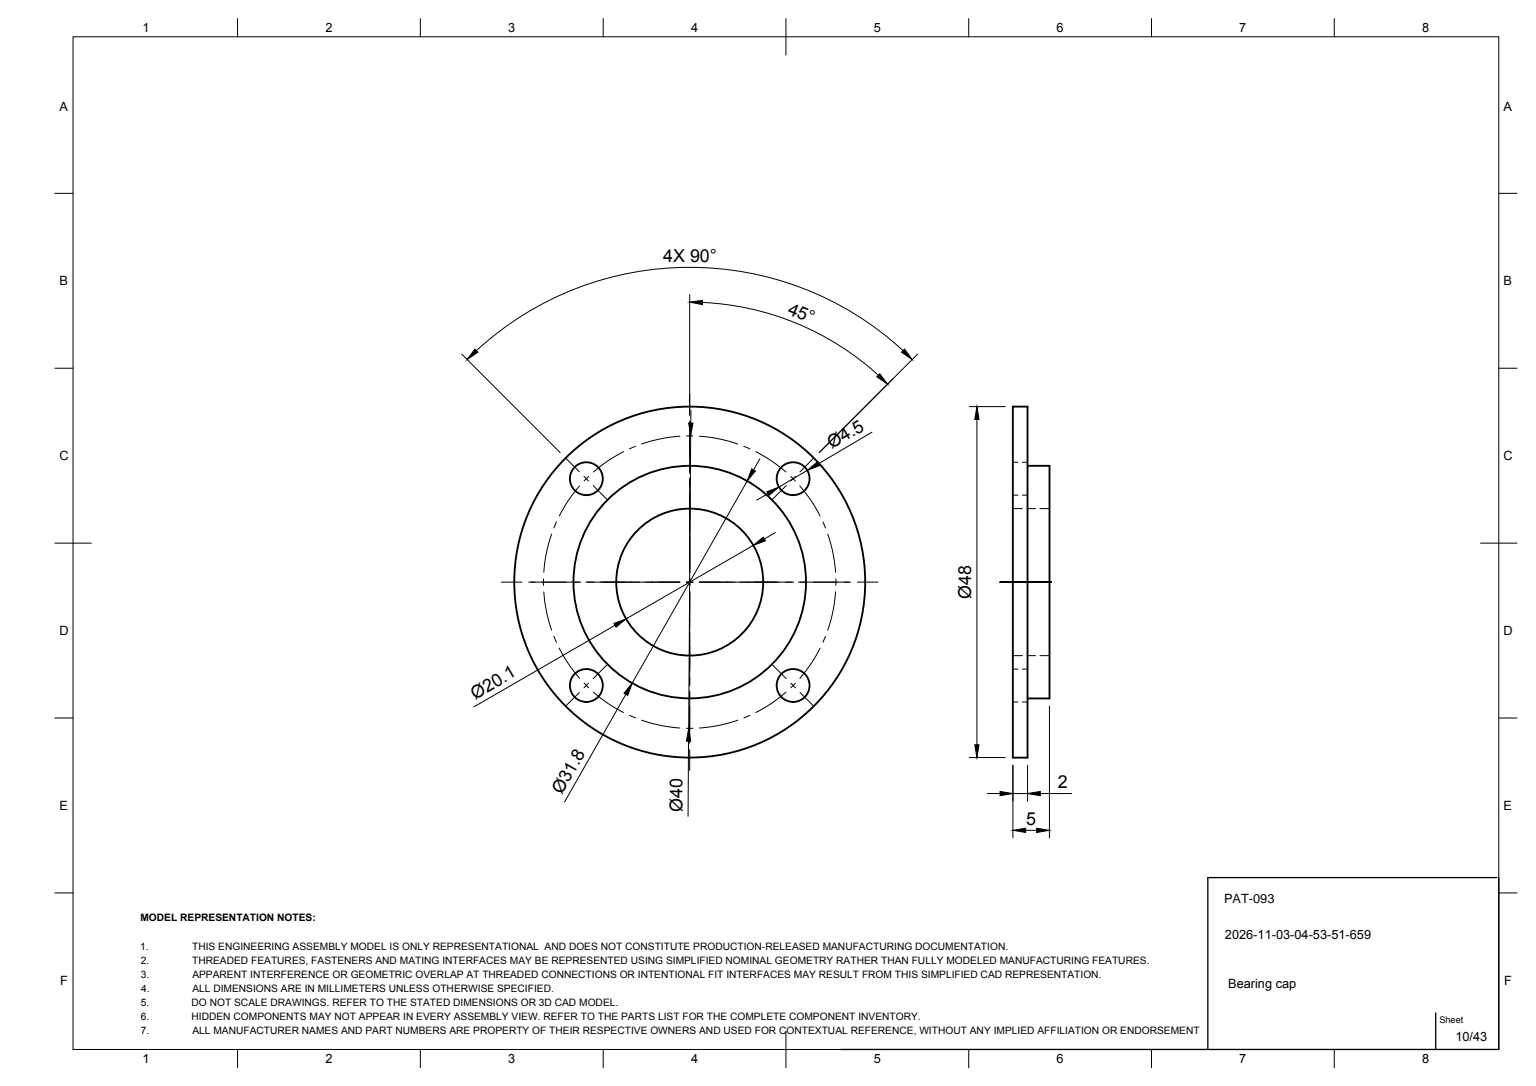
ISO-10303-21;
HEADER;
/* Generated by software containing ST-Developer
 * from STEP Tools, Inc. (www.steptools.com) 
 */

FILE_DESCRIPTION(
/* description */ ('Self-centering screw clamp'),
/* implementation_level */ '2;1');

FILE_NAME(
/* name */ 'Bearing cap.step',
/* time_stamp */ '2026-10-28T03:25:31-07:00',
/* author */ (''),
/* organization */ (''),
/* preprocessor_version */ 'ST-DEVELOPER v20.2',
/* originating_system */ 'Autodesk Translation Framework v15.17.0.0',
/* authorisation */ '');

FILE_SCHEMA (('AUTOMOTIVE_DESIGN { 1 0 10303 214 3 1 1 }'));
ENDSEC;

DATA;
#10=MECHANICAL_DESIGN_GEOMETRIC_PRESENTATION_REPRESENTATION('',(#632),#16799);
#550=SHAPE_REPRESENTATION_RELATIONSHIP('SRR','None',#17023,#591);
#591=ADVANCED_BREP_SHAPE_REPRESENTATION('',(#680),#16761);
#632=STYLED_ITEM('',(#17326),#680);
#680=MANIFOLD_SOLID_BREP('Body1',#9083);
#784=FACE_BOUND('',#1968,.T.);
#785=FACE_BOUND('',#1972,.T.);
#786=FACE_BOUND('',#1973,.T.);
#787=FACE_BOUND('',#1974,.T.);
#788=FACE_BOUND('',#1975,.T.);
#789=FACE_BOUND('',#1976,.T.);
#790=FACE_BOUND('',#1978,.T.);
#791=FACE_BOUND('',#1979,.T.);
#792=FACE_BOUND('',#1980,.T.);
#793=FACE_BOUND('',#1981,.T.);
#794=FACE_BOUND('',#1982,.T.);
#1082=PLANE('',#9828);
#1083=PLANE('',#9835);
#1084=PLANE('',#9836);
#1392=FACE_OUTER_BOUND('',#1962,.T.);
#1393=FACE_OUTER_BOUND('',#1963,.T.);
#1394=FACE_OUTER_BOUND('',#1964,.T.);
#1395=FACE_OUTER_BOUND('',#1965,.T.);
#1396=FACE_OUTER_BOUND('',#1966,.T.);
#1397=FACE_OUTER_BOUND('',#1967,.T.);
#1398=FACE_OUTER_BOUND('',#1969,.T.);
#1399=FACE_OUTER_BOUND('',#1970,.T.);
#1400=FACE_OUTER_BOUND('',#1971,.T.);
#1401=FACE_OUTER_BOUND('',#1977,.T.);
#1962=EDGE_LOOP('',(#6721,#6722,#6723,#6724));
#1963=EDGE_LOOP('',(#6725,#6726,#6727,#6728));
#1964=EDGE_LOOP('',(#6729,#6730,#6731,#6732));
#1965=EDGE_LOOP('',(#6733,#6734,#6735,#6736));
#1966=EDGE_LOOP('',(#6737,#6738,#6739,#6740));
#1967=EDGE_LOOP('',(#6741));
#1968=EDGE_LOOP('',(#6742));
#1969=EDGE_LOOP('',(#6743,#6744,#6745,#6746));
#1970=EDGE_LOOP('',(#6747,#6748,#6749,#6750));
#1971=EDGE_LOOP('',(#6751));
#1972=EDGE_LOOP('',(#6752));
#1973=EDGE_LOOP('',(#6753));
#1974=EDGE_LOOP('',(#6754));
#1975=EDGE_LOOP('',(#6755));
#1976=EDGE_LOOP('',(#6756));
#1977=EDGE_LOOP('',(#6757));
#1978=EDGE_LOOP('',(#6758));
#1979=EDGE_LOOP('',(#6759));
#1980=EDGE_LOOP('',(#6760));
#1981=EDGE_LOOP('',(#6761));
#1982=EDGE_LOOP('',(#6762));
#2764=LINE('',#14392,#3337);
#2765=LINE('',#14398,#3338);
#2766=LINE('',#14404,#3339);
#2767=LINE('',#14410,#3340);
#2768=LINE('',#14416,#3341);
#2769=LINE('',#14423,#3342);
#2770=LINE('',#14429,#3343);
#3337=VECTOR('',#11415,0.225);
#3338=VECTOR('',#11422,0.225);
#3339=VECTOR('',#11429,0.225);
#3340=VECTOR('',#11436,0.225);
#3341=VECTOR('',#11443,1.59);
#3342=VECTOR('',#11452,1.005);
#3343=VECTOR('',#11459,2.4);
#3829=CIRCLE('',#9814,0.225);
#3830=CIRCLE('',#9815,0.225);
#3831=CIRCLE('',#9817,0.225);
#3832=CIRCLE('',#9818,0.225);
#3833=CIRCLE('',#9820,0.225);
#3834=CIRCLE('',#9821,0.225);
#3835=CIRCLE('',#9823,0.225);
#3836=CIRCLE('',#9824,0.225);
#3837=CIRCLE('',#9826,1.59);
#3838=CIRCLE('',#9827,1.59);
#3839=CIRCLE('',#9829,1.005);
#3840=CIRCLE('',#9831,1.005);
#3841=CIRCLE('',#9833,2.4);
#3842=CIRCLE('',#9834,2.4);
#4427=VERTEX_POINT('',#14389);
#4428=VERTEX_POINT('',#14391);
#4429=VERTEX_POINT('',#14395);
#4430=VERTEX_POINT('',#14397);
#4431=VERTEX_POINT('',#14401);
#4432=VERTEX_POINT('',#14403);
#4433=VERTEX_POINT('',#14407);
#4434=VERTEX_POINT('',#14409);
#4435=VERTEX_POINT('',#14413);
#4436=VERTEX_POINT('',#14415);
#4437=VERTEX_POINT('',#14419);
#4438=VERTEX_POINT('',#14422);
#4439=VERTEX_POINT('',#14426);
#4440=VERTEX_POINT('',#14428);
#5285=EDGE_CURVE('',#4427,#4427,#3829,.T.);
#5286=EDGE_CURVE('',#4427,#4428,#2764,.T.);
#5287=EDGE_CURVE('',#4428,#4428,#3830,.T.);
#5288=EDGE_CURVE('',#4429,#4429,#3831,.T.);
#5289=EDGE_CURVE('',#4429,#4430,#2765,.T.);
#5290=EDGE_CURVE('',#4430,#4430,#3832,.T.);
#5291=EDGE_CURVE('',#4431,#4431,#3833,.T.);
#5292=EDGE_CURVE('',#4431,#4432,#2766,.T.);
#5293=EDGE_CURVE('',#4432,#4432,#3834,.T.);
#5294=EDGE_CURVE('',#4433,#4433,#3835,.T.);
#5295=EDGE_CURVE('',#4433,#4434,#2767,.T.);
#5296=EDGE_CURVE('',#4434,#4434,#3836,.T.);
#5297=EDGE_CURVE('',#4435,#4435,#3837,.T.);
#5298=EDGE_CURVE('',#4435,#4436,#2768,.T.);
#5299=EDGE_CURVE('',#4436,#4436,#3838,.T.);
#5300=EDGE_CURVE('',#4437,#4437,#3839,.T.);
#5301=EDGE_CURVE('',#4437,#4438,#2769,.T.);
#5302=EDGE_CURVE('',#4438,#4438,#3840,.T.);
#5303=EDGE_CURVE('',#4439,#4439,#3841,.T.);
#5304=EDGE_CURVE('',#4439,#4440,#2770,.T.);
#5305=EDGE_CURVE('',#4440,#4440,#3842,.T.);
#6721=ORIENTED_EDGE('',*,*,#5285,.F.);
#6722=ORIENTED_EDGE('',*,*,#5286,.T.);
#6723=ORIENTED_EDGE('',*,*,#5287,.F.);
#6724=ORIENTED_EDGE('',*,*,#5286,.F.);
#6725=ORIENTED_EDGE('',*,*,#5288,.F.);
#6726=ORIENTED_EDGE('',*,*,#5289,.T.);
#6727=ORIENTED_EDGE('',*,*,#5290,.F.);
#6728=ORIENTED_EDGE('',*,*,#5289,.F.);
#6729=ORIENTED_EDGE('',*,*,#5291,.F.);
#6730=ORIENTED_EDGE('',*,*,#5292,.T.);
#6731=ORIENTED_EDGE('',*,*,#5293,.F.);
#6732=ORIENTED_EDGE('',*,*,#5292,.F.);
#6733=ORIENTED_EDGE('',*,*,#5294,.F.);
#6734=ORIENTED_EDGE('',*,*,#5295,.T.);
#6735=ORIENTED_EDGE('',*,*,#5296,.F.);
#6736=ORIENTED_EDGE('',*,*,#5295,.F.);
#6737=ORIENTED_EDGE('',*,*,#5297,.F.);
#6738=ORIENTED_EDGE('',*,*,#5298,.T.);
#6739=ORIENTED_EDGE('',*,*,#5299,.F.);
#6740=ORIENTED_EDGE('',*,*,#5298,.F.);
#6741=ORIENTED_EDGE('',*,*,#5297,.T.);
#6742=ORIENTED_EDGE('',*,*,#5300,.T.);
#6743=ORIENTED_EDGE('',*,*,#5300,.F.);
#6744=ORIENTED_EDGE('',*,*,#5301,.T.);
#6745=ORIENTED_EDGE('',*,*,#5302,.T.);
#6746=ORIENTED_EDGE('',*,*,#5301,.F.);
#6747=ORIENTED_EDGE('',*,*,#5303,.F.);
#6748=ORIENTED_EDGE('',*,*,#5304,.T.);
#6749=ORIENTED_EDGE('',*,*,#5305,.T.);
#6750=ORIENTED_EDGE('',*,*,#5304,.F.);
#6751=ORIENTED_EDGE('',*,*,#5303,.T.);
#6752=ORIENTED_EDGE('',*,*,#5299,.T.);
#6753=ORIENTED_EDGE('',*,*,#5296,.T.);
#6754=ORIENTED_EDGE('',*,*,#5293,.T.);
#6755=ORIENTED_EDGE('',*,*,#5290,.T.);
#6756=ORIENTED_EDGE('',*,*,#5287,.T.);
#6757=ORIENTED_EDGE('',*,*,#5305,.F.);
#6758=ORIENTED_EDGE('',*,*,#5302,.F.);
#6759=ORIENTED_EDGE('',*,*,#5294,.T.);
#6760=ORIENTED_EDGE('',*,*,#5291,.T.);
#6761=ORIENTED_EDGE('',*,*,#5288,.T.);
#6762=ORIENTED_EDGE('',*,*,#5285,.T.);
#8408=CYLINDRICAL_SURFACE('',#9813,0.225);
#8409=CYLINDRICAL_SURFACE('',#9816,0.225);
#8410=CYLINDRICAL_SURFACE('',#9819,0.225);
#8411=CYLINDRICAL_SURFACE('',#9822,0.225);
#8412=CYLINDRICAL_SURFACE('',#9825,1.59);
#8413=CYLINDRICAL_SURFACE('',#9830,1.005);
#8414=CYLINDRICAL_SURFACE('',#9832,2.4);
#8690=ADVANCED_FACE('',(#1392),#8408,.F.);
#8691=ADVANCED_FACE('',(#1393),#8409,.F.);
#8692=ADVANCED_FACE('',(#1394),#8410,.F.);
#8693=ADVANCED_FACE('',(#1395),#8411,.F.);
#8694=ADVANCED_FACE('',(#1396),#8412,.T.);
#8695=ADVANCED_FACE('',(#1397,#784),#1082,.T.);
#8696=ADVANCED_FACE('',(#1398),#8413,.F.);
#8697=ADVANCED_FACE('',(#1399),#8414,.T.);
#8698=ADVANCED_FACE('',(#1400,#785,#786,#787,#788,#789),#1083,.T.);
#8699=ADVANCED_FACE('',(#1401,#790,#791,#792,#793,#794),#1084,.F.);
#9083=CLOSED_SHELL('',(#8690,#8691,#8692,#8693,#8694,#8695,#8696,#8697,
#8698,#8699));
#9812=AXIS2_PLACEMENT_3D('',#14387,#11409,#11410);
#9813=AXIS2_PLACEMENT_3D('',#14388,#11411,#11412);
#9814=AXIS2_PLACEMENT_3D('',#14390,#11413,#11414);
#9815=AXIS2_PLACEMENT_3D('',#14393,#11416,#11417);
#9816=AXIS2_PLACEMENT_3D('',#14394,#11418,#11419);
#9817=AXIS2_PLACEMENT_3D('',#14396,#11420,#11421);
#9818=AXIS2_PLACEMENT_3D('',#14399,#11423,#11424);
#9819=AXIS2_PLACEMENT_3D('',#14400,#11425,#11426);
#9820=AXIS2_PLACEMENT_3D('',#14402,#11427,#11428);
#9821=AXIS2_PLACEMENT_3D('',#14405,#11430,#11431);
#9822=AXIS2_PLACEMENT_3D('',#14406,#11432,#11433);
#9823=AXIS2_PLACEMENT_3D('',#14408,#11434,#11435);
#9824=AXIS2_PLACEMENT_3D('',#14411,#11437,#11438);
#9825=AXIS2_PLACEMENT_3D('',#14412,#11439,#11440);
#9826=AXIS2_PLACEMENT_3D('',#14414,#11441,#11442);
#9827=AXIS2_PLACEMENT_3D('',#14417,#11444,#11445);
#9828=AXIS2_PLACEMENT_3D('',#14418,#11446,#11447);
#9829=AXIS2_PLACEMENT_3D('',#14420,#11448,#11449);
#9830=AXIS2_PLACEMENT_3D('',#14421,#11450,#11451);
#9831=AXIS2_PLACEMENT_3D('',#14424,#11453,#11454);
#9832=AXIS2_PLACEMENT_3D('',#14425,#11455,#11456);
#9833=AXIS2_PLACEMENT_3D('',#14427,#11457,#11458);
#9834=AXIS2_PLACEMENT_3D('',#14430,#11460,#11461);
#9835=AXIS2_PLACEMENT_3D('',#14431,#11462,#11463);
#9836=AXIS2_PLACEMENT_3D('',#14432,#11464,#11465);
#11409=DIRECTION('axis',(0.,0.,1.));
#11410=DIRECTION('refdir',(1.,0.,0.));
#11411=DIRECTION('center_axis',(1.,0.,0.));
#11412=DIRECTION('ref_axis',(0.,0.,-1.));
#11413=DIRECTION('center_axis',(1.,0.,0.));
#11414=DIRECTION('ref_axis',(0.,0.,-1.));
#11415=DIRECTION('',(1.,0.,0.));
#11416=DIRECTION('center_axis',(-1.,0.,0.));
#11417=DIRECTION('ref_axis',(0.,0.,-1.));
#11418=DIRECTION('center_axis',(1.,0.,0.));
#11419=DIRECTION('ref_axis',(0.,0.,-1.));
#11420=DIRECTION('center_axis',(1.,0.,0.));
#11421=DIRECTION('ref_axis',(0.,0.,-1.));
#11422=DIRECTION('',(1.,0.,0.));
#11423=DIRECTION('center_axis',(-1.,0.,0.));
#11424=DIRECTION('ref_axis',(0.,0.,-1.));
#11425=DIRECTION('center_axis',(1.,0.,0.));
#11426=DIRECTION('ref_axis',(0.,0.,-1.));
#11427=DIRECTION('center_axis',(1.,0.,0.));
#11428=DIRECTION('ref_axis',(0.,0.,-1.));
#11429=DIRECTION('',(1.,0.,0.));
#11430=DIRECTION('center_axis',(-1.,0.,0.));
#11431=DIRECTION('ref_axis',(0.,0.,-1.));
#11432=DIRECTION('center_axis',(1.,0.,0.));
#11433=DIRECTION('ref_axis',(0.,0.,-1.));
#11434=DIRECTION('center_axis',(1.,0.,0.));
#11435=DIRECTION('ref_axis',(0.,0.,-1.));
#11436=DIRECTION('',(1.,0.,0.));
#11437=DIRECTION('center_axis',(-1.,0.,0.));
#11438=DIRECTION('ref_axis',(0.,0.,-1.));
#11439=DIRECTION('center_axis',(1.,0.,0.));
#11440=DIRECTION('ref_axis',(0.,0.,-1.));
#11441=DIRECTION('center_axis',(1.,0.,0.));
#11442=DIRECTION('ref_axis',(0.,0.,-1.));
#11443=DIRECTION('',(-1.,0.,0.));
#11444=DIRECTION('center_axis',(-1.,0.,0.));
#11445=DIRECTION('ref_axis',(0.,0.,-1.));
#11446=DIRECTION('center_axis',(1.,0.,0.));
#11447=DIRECTION('ref_axis',(0.,0.,-1.));
#11448=DIRECTION('center_axis',(-1.,0.,0.));
#11449=DIRECTION('ref_axis',(0.,0.,-1.));
#11450=DIRECTION('center_axis',(1.,0.,0.));
#11451=DIRECTION('ref_axis',(0.,0.,-1.));
#11452=DIRECTION('',(-1.,0.,0.));
#11453=DIRECTION('center_axis',(-1.,0.,0.));
#11454=DIRECTION('ref_axis',(0.,0.,-1.));
#11455=DIRECTION('center_axis',(1.,0.,0.));
#11456=DIRECTION('ref_axis',(0.,0.,-1.));
#11457=DIRECTION('center_axis',(1.,0.,0.));
#11458=DIRECTION('ref_axis',(0.,0.,-1.));
#11459=DIRECTION('',(-1.,0.,0.));
#11460=DIRECTION('center_axis',(1.,0.,0.));
#11461=DIRECTION('ref_axis',(0.,0.,-1.));
#11462=DIRECTION('center_axis',(1.,0.,0.));
#11463=DIRECTION('ref_axis',(0.,0.,-1.));
#11464=DIRECTION('center_axis',(1.,0.,0.));
#11465=DIRECTION('ref_axis',(0.,0.,-1.));
#14387=CARTESIAN_POINT('',(0.,0.,0.));
#14388=CARTESIAN_POINT('Origin',(-12.6,-1.4142135623731,2.58578643762691));
#14389=CARTESIAN_POINT('',(-12.5,-1.4142135623731,2.81078643762691));
#14390=CARTESIAN_POINT('Origin',(-12.5,-1.4142135623731,2.58578643762691));
#14391=CARTESIAN_POINT('',(-12.3,-1.4142135623731,2.81078643762691));
#14392=CARTESIAN_POINT('',(-12.6,-1.4142135623731,2.81078643762691));
#14393=CARTESIAN_POINT('Origin',(-12.3,-1.4142135623731,2.58578643762691));
#14394=CARTESIAN_POINT('Origin',(-12.6,-1.41421356237309,5.41421356237309));
#14395=CARTESIAN_POINT('',(-12.5,-1.41421356237309,5.63921356237309));
#14396=CARTESIAN_POINT('Origin',(-12.5,-1.41421356237309,5.41421356237309));
#14397=CARTESIAN_POINT('',(-12.3,-1.41421356237309,5.63921356237309));
#14398=CARTESIAN_POINT('',(-12.6,-1.41421356237309,5.63921356237309));
#14399=CARTESIAN_POINT('Origin',(-12.3,-1.41421356237309,5.41421356237309));
#14400=CARTESIAN_POINT('Origin',(-12.6,1.4142135623731,5.41421356237309));
#14401=CARTESIAN_POINT('',(-12.5,1.4142135623731,5.63921356237309));
#14402=CARTESIAN_POINT('Origin',(-12.5,1.4142135623731,5.41421356237309));
#14403=CARTESIAN_POINT('',(-12.3,1.4142135623731,5.63921356237309));
#14404=CARTESIAN_POINT('',(-12.6,1.4142135623731,5.63921356237309));
#14405=CARTESIAN_POINT('Origin',(-12.3,1.4142135623731,5.41421356237309));
#14406=CARTESIAN_POINT('Origin',(-12.6,1.41421356237309,2.5857864376269));
#14407=CARTESIAN_POINT('',(-12.5,1.41421356237309,2.8107864376269));
#14408=CARTESIAN_POINT('Origin',(-12.5,1.41421356237309,2.5857864376269));
#14409=CARTESIAN_POINT('',(-12.3,1.41421356237309,2.8107864376269));
#14410=CARTESIAN_POINT('',(-12.6,1.41421356237309,2.8107864376269));
#14411=CARTESIAN_POINT('Origin',(-12.3,1.41421356237309,2.5857864376269));
#14412=CARTESIAN_POINT('Origin',(-12.3,0.,4.));
#14413=CARTESIAN_POINT('',(-12.,-1.94718841064429E-16,5.59));
#14414=CARTESIAN_POINT('Origin',(-12.,0.,4.));
#14415=CARTESIAN_POINT('',(-12.3,-1.94718841064429E-16,5.59));
#14416=CARTESIAN_POINT('',(-12.3,-1.94718841064429E-16,5.59));
#14417=CARTESIAN_POINT('Origin',(-12.3,0.,4.));
#14418=CARTESIAN_POINT('Origin',(-12.,0.,4.));
#14419=CARTESIAN_POINT('',(-12.,-1.23077003314309E-16,5.005));
#14420=CARTESIAN_POINT('Origin',(-12.,0.,4.));
#14421=CARTESIAN_POINT('Origin',(-12.5,0.,4.));
#14422=CARTESIAN_POINT('',(-12.5,-1.23077003314309E-16,5.005));
#14423=CARTESIAN_POINT('',(-12.5,-1.23077003314309E-16,5.005));
#14424=CARTESIAN_POINT('Origin',(-12.5,0.,4.));
#14425=CARTESIAN_POINT('Origin',(-12.5,0.,4.));
#14426=CARTESIAN_POINT('',(-12.3,-2.93915231795365E-16,6.4));
#14427=CARTESIAN_POINT('Origin',(-12.3,0.,4.));
#14428=CARTESIAN_POINT('',(-12.5,-2.93915231795365E-16,6.4));
#14429=CARTESIAN_POINT('',(-12.5,-2.93915231795365E-16,6.4));
#14430=CARTESIAN_POINT('Origin',(-12.5,0.,4.));
#14431=CARTESIAN_POINT('Origin',(-12.3,0.,4.));
#14432=CARTESIAN_POINT('Origin',(-12.5,0.,4.));
#16712=UNCERTAINTY_MEASURE_WITH_UNIT(LENGTH_MEASURE(0.001),#16800,
'DISTANCE_ACCURACY_VALUE',
'Maximum model space distance between geometric entities at asserted c
onnectivities');
#16750=UNCERTAINTY_MEASURE_WITH_UNIT(LENGTH_MEASURE(0.001),#16800,
'DISTANCE_ACCURACY_VALUE',
'Maximum model space distance between geometric entities at asserted c
onnectivities');
#16761=(
GEOMETRIC_REPRESENTATION_CONTEXT(3)
GLOBAL_UNCERTAINTY_ASSIGNED_CONTEXT((#16712))
GLOBAL_UNIT_ASSIGNED_CONTEXT((#16800,#16802,#16803))
REPRESENTATION_CONTEXT('','3D')
);
#16799=(
GEOMETRIC_REPRESENTATION_CONTEXT(3)
GLOBAL_UNCERTAINTY_ASSIGNED_CONTEXT((#16750))
GLOBAL_UNIT_ASSIGNED_CONTEXT((#16800,#16802,#16803))
REPRESENTATION_CONTEXT('','3D')
);
#16800=(
LENGTH_UNIT()
NAMED_UNIT(*)
SI_UNIT(.CENTI.,.METRE.)
);
#16802=(
NAMED_UNIT(*)
PLANE_ANGLE_UNIT()
SI_UNIT($,.RADIAN.)
);
#16803=(
NAMED_UNIT(*)
SI_UNIT($,.STERADIAN.)
SOLID_ANGLE_UNIT()
);
#16814=SHAPE_DEFINITION_REPRESENTATION(#16862,#17023);
#16862=PRODUCT_DEFINITION_SHAPE('',$,#17072);
#17023=SHAPE_REPRESENTATION('',(#9812),#16761);
#17061=PRODUCT_DEFINITION_CONTEXT('part definition',#17207,'design');
#17072=PRODUCT_DEFINITION('Bearing cap','Bearing cap',#17120,#17061);
#17120=PRODUCT_DEFINITION_FORMATION('',$,#17219);
#17207=APPLICATION_CONTEXT(
'Core Data for Automotive Mechanical Design Process');
#17208=PRODUCT_CONTEXT('part definition',#17207,'mechanical');
#17219=PRODUCT('Bearing cap','Bearing cap','Bearing cap',(#17208));
#17320=COLOUR_RGB('Grey',0.48,0.52,0.57);
#17321=FILL_AREA_STYLE_COLOUR('',#17320);
#17322=FILL_AREA_STYLE('',(#17321));
#17323=SURFACE_STYLE_FILL_AREA(#17322);
#17324=SURFACE_SIDE_STYLE('',(#17323));
#17325=SURFACE_STYLE_USAGE(.BOTH.,#17324);
#17326=PRESENTATION_STYLE_ASSIGNMENT((#17325));
ENDSEC;
END-ISO-10303-21;
